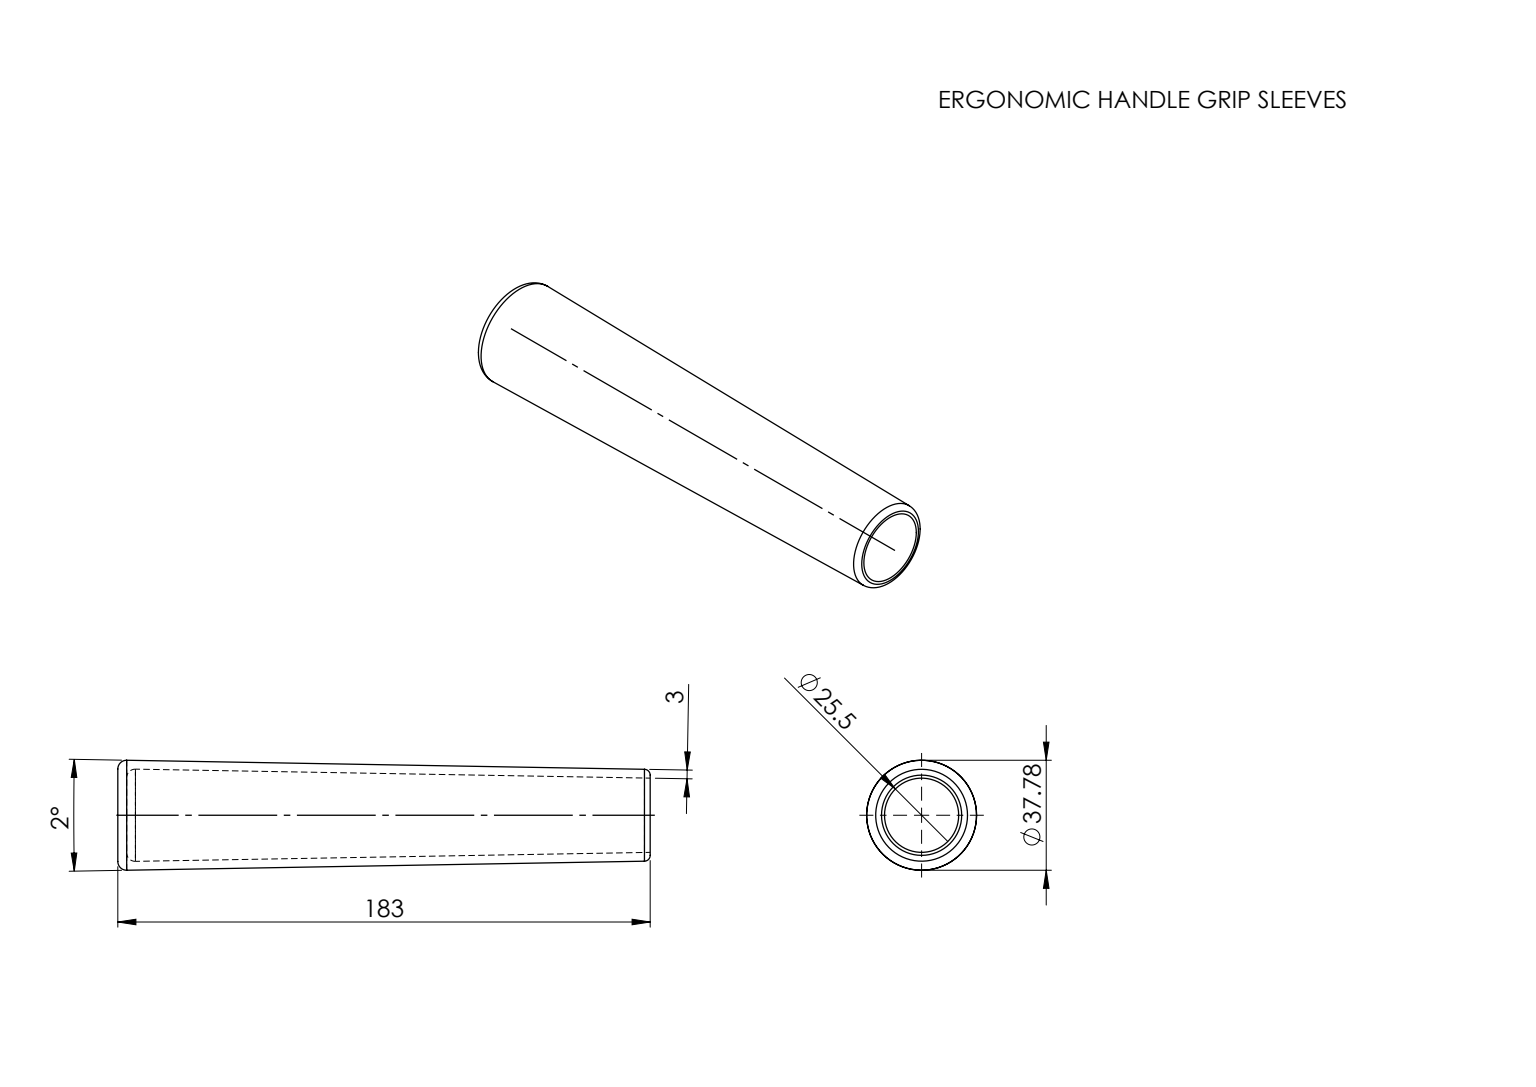
ISO-10303-21;
HEADER;
FILE_DESCRIPTION (('STEP AP214'),
    '1' );
FILE_NAME ('Ergonomic Handle Grip Sleeves.step',
    '2026-10-02T13:02:33',
    ( '' ),
    ( '' ),
    'SwSTEP 2.0',
    'SolidWorks 2026',
    '' );
FILE_SCHEMA (( 'AUTOMOTIVE_DESIGN' ));
ENDSEC;

DATA;
#12=AXIS2_PLACEMENT_3D ( 'NONE', #5144, #6683, #9508 ) ;
#70=( NAMED_UNIT ( * ) SI_UNIT ( $, .STERADIAN. ) SOLID_ANGLE_UNIT ( ) );
#80=ORIENTED_EDGE ( 'NONE', *, *, #17512, .T. ) ;
#102=ORIENTED_EDGE ( 'NONE', *, *, #16935, .T. ) ;
#181=ORIENTED_EDGE ( 'NONE', *, *, #3310, .F. ) ;
#194=( NAMED_UNIT ( * ) PLANE_ANGLE_UNIT ( ) SI_UNIT ( $, .RADIAN. ) );
#220=EDGE_CURVE ( 'NONE', #5802, #9058, #10861, .T. ) ;
#233=ORIENTED_EDGE ( 'NONE', *, *, #9764, .F. ) ;
#364=APPLICATION_CONTEXT ( 'automotive_design' ) ;
#380=CIRCLE ( 'NONE', #16419, 13.78215425775057668 ) ;
#447=DIRECTION ( 'NONE',  ( 0.000000000000000000, 0.000000000000000000, -1.000000000000000000 ) ) ;
#481=CARTESIAN_POINT ( 'NONE',  ( -131.1404785418517918, -2.850701963179328668, -13.78215425775057490 ) ) ;
#490=CIRCLE ( 'NONE', #15932, 13.78215425775057668 ) ;
#611=FACE_OUTER_BOUND ( 'NONE', #2046, .T. ) ;
#789=CARTESIAN_POINT ( 'NONE',  ( -131.1055737289773617, -2.850701963179328668, 9.951701414186818625E-16 ) ) ;
#845=ORIENTED_EDGE ( 'NONE', *, *, #9764, .T. ) ;
#922=CARTESIAN_POINT ( 'NONE',  ( -129.1404785418517918, -2.850701963179328668, 9.951701414186818625E-16 ) ) ;
#1010=ORIENTED_EDGE ( 'NONE', *, *, #8263, .T. ) ;
#1036=EDGE_LOOP ( 'NONE', ( #5576, #5988 ) ) ;
#1053=ORIENTED_EDGE ( 'NONE', *, *, #2494, .F. ) ;
#1132=VERTEX_POINT ( 'NONE', #18787 ) ;
#1237=ORIENTED_EDGE ( 'NONE', *, *, #1546, .T. ) ;
#1428=DIRECTION ( 'NONE',  ( 0.000000000000000000, 0.000000000000000000, 1.000000000000000000 ) ) ;
#1519=CARTESIAN_POINT ( 'NONE',  ( -306.0881213225399051, -2.850701963179328668, 9.951701414186818625E-16 ) ) ;
#1525=CIRCLE ( 'NONE', #11179, 18.88854657239857815 ) ;
#1546=EDGE_CURVE ( 'NONE', #6009, #3698, #17797, .T. ) ;
#1589=( NAMED_UNIT ( * ) PLANE_ANGLE_UNIT ( ) SI_UNIT ( $, .RADIAN. ) );
#1674=DIRECTION ( 'NONE',  ( -1.000000000000000000, 0.000000000000000000, 0.000000000000000000 ) ) ;
#1677=EDGE_LOOP ( 'NONE', ( #11273, #1237, #15915, #6184 ) ) ;
#1683=DIRECTION ( 'NONE',  ( 0.000000000000000000, 1.000000000000000000, -1.224646799147353207E-16 ) ) ;
#1701=ORIENTED_EDGE ( 'NONE', *, *, #4888, .T. ) ;
#1709=ORIENTED_EDGE ( 'NONE', *, *, #10798, .T. ) ;
#1812=FACE_OUTER_BOUND ( 'NONE', #16311, .T. ) ;
#1827=CIRCLE ( 'NONE', #14256, 18.88854657239857815 ) ;
#1899=UNCERTAINTY_MEASURE_WITH_UNIT (LENGTH_MEASURE( 1.000000000000000082E-05 ), #7601, 'distance_accuracy_value', 'NONE');
#1933=EDGE_CURVE ( 'NONE', #6009, #10091, #5194, .T. ) ;
#2046=EDGE_LOOP ( 'NONE', ( #7736, #9894, #11498, #9115 ) ) ;
#2058=CARTESIAN_POINT ( 'NONE',  ( -129.1404785418517918, -2.850701963179328668, 9.951701414186818625E-16 ) ) ;
#2108=CARTESIAN_POINT ( 'NONE',  ( -309.1404785418517918, -2.850701963179328668, 9.951701414186818625E-16 ) ) ;
#2162=DIRECTION ( 'NONE',  ( 0.000000000000000000, 0.000000000000000000, -1.000000000000000000 ) ) ;
#2247=DIRECTION ( 'NONE',  ( 0.000000000000000000, -1.000000000000000000, 0.000000000000000000 ) ) ;
#2480=MANIFOLD_SOLID_BREP ( 'Cavity1', #10549 ) ;
#2486=ORIENTED_EDGE ( 'NONE', *, *, #10798, .F. ) ;
#2487=ADVANCED_FACE ( 'NONE', ( #1812 ), #4558, .T. ) ;
#2489=EDGE_CURVE ( 'NONE', #6795, #5802, #5832, .T. ) ;
#2494=EDGE_CURVE ( 'NONE', #10067, #10091, #380, .T. ) ;
#2512=CARTESIAN_POINT ( 'NONE',  ( -131.1055737289773617, -2.850701963179328668, -15.78184964806336055 ) ) ;
#2533=DIRECTION ( 'NONE',  ( -1.000000000000000000, 0.000000000000000000, 0.000000000000000000 ) ) ;
#2537=VERTEX_POINT ( 'NONE', #10885 ) ;
#2720=CARTESIAN_POINT ( 'NONE',  ( -309.1404785418517918, -2.850701963179328668, 9.951701414186818625E-16 ) ) ;
#2763=VECTOR ( 'NONE', #3525, 1000.000000000000114 ) ;
#2778=CARTESIAN_POINT ( 'NONE',  ( -129.1404785418517918, -2.850701963179326892, -12.74754878398196389 ) ) ;
#2882=EDGE_CURVE ( 'NONE', #3698, #9058, #7770, .T. ) ;
#2886=( NAMED_UNIT ( * ) SI_UNIT ( $, .STERADIAN. ) SOLID_ANGLE_UNIT ( ) );
#2950=EDGE_LOOP ( 'NONE', ( #7070, #12584, #14818, #11398 ) ) ;
#2982=FACE_OUTER_BOUND ( 'NONE', #15483, .T. ) ;
#3054=CARTESIAN_POINT ( 'NONE',  ( -129.1404785418517918, -2.850701963179328668, 9.951701414186818625E-16 ) ) ;
#3061=ADVANCED_FACE ( 'NONE', ( #11418 ), #3510, .T. ) ;
#3149=ORIENTED_EDGE ( 'NONE', *, *, #17512, .F. ) ;
#3162=DIRECTION ( 'NONE',  ( -1.000000000000000000, 0.000000000000000000, 0.000000000000000000 ) ) ;
#3182=DIRECTION ( 'NONE',  ( -0.9998476951563911586, 0.000000000000000000, 0.01745240643728354635 ) ) ;
#3210=PRESENTATION_STYLE_ASSIGNMENT (( #14519 ) ) ;
#3227=VERTEX_POINT ( 'NONE', #4413 ) ;
#3262=CONICAL_SURFACE ( 'NONE', #5717, 15.74754878398195856, 0.01745329251994333364 ) ;
#3285=CARTESIAN_POINT ( 'NONE',  ( -129.1404785418517918, -2.850701963179328668, 9.951701414186818625E-16 ) ) ;
#3310=EDGE_CURVE ( 'NONE', #2537, #8740, #16558, .T. ) ;
#3339=CARTESIAN_POINT ( 'NONE',  ( -129.1404785418517918, -2.850701963179328668, 9.951701414186818625E-16 ) ) ;
#3365=AXIS2_PLACEMENT_3D ( 'NONE', #3054, #11477, #14434 ) ;
#3397=CARTESIAN_POINT ( 'NONE',  ( -129.1404785418517918, -2.850701963179328668, 9.951701414186818625E-16 ) ) ;
#3510=TOROIDAL_SURFACE ( 'NONE', #12607, 13.78215425775057668, 2.000000000000000000 ) ;
#3525=DIRECTION ( 'NONE',  ( -0.9998476951563911586, -2.137303368083795934E-18, 0.01745240643728354635 ) ) ;
#3566=ORIENTED_EDGE ( 'NONE', *, *, #18340, .F. ) ;
#3571=CARTESIAN_POINT ( 'NONE',  ( -312.1404785418517918, -2.850701963179328668, 15.88900348692940945 ) ) ;
#3616=CONICAL_SURFACE ( 'NONE', #14826, 12.74754878398196567, 0.01745329251994333364 ) ;
#3698=VERTEX_POINT ( 'NONE', #6213 ) ;
#3713=CARTESIAN_POINT ( 'NONE',  ( -309.1404785418517918, -2.850701963179328668, 9.951701414186818625E-16 ) ) ;
#3936=PRODUCT ( 'Ergonomic Handle Grip Sleeves', 'Ergonomic Handle Grip Sleeves', '', ( #17404 ) ) ;
#4038=ADVANCED_FACE ( 'NONE', ( #11937 ), #3616, .F. ) ;
#4042=EDGE_CURVE ( 'NONE', #10626, #3227, #8172, .T. ) ;
#4073=ORIENTED_EDGE ( 'NONE', *, *, #9817, .T. ) ;
#4106=DIRECTION ( 'NONE',  ( 0.000000000000000000, 0.000000000000000000, -1.000000000000000000 ) ) ;
#4113=AXIS2_PLACEMENT_3D ( 'NONE', #14799, #7611, #12017 ) ;
#4153=DIRECTION ( 'NONE',  ( -1.000000000000000000, 0.000000000000000000, 0.000000000000000000 ) ) ;
#4207=EDGE_CURVE ( 'NONE', #6795, #3698, #1827, .T. ) ;
#4223=SURFACE_STYLE_FILL_AREA ( #9827 ) ;
#4381=DIRECTION ( 'NONE',  ( 0.000000000000000000, 1.000000000000000000, 1.224646799147353207E-16 ) ) ;
#4413=CARTESIAN_POINT ( 'NONE',  ( -309.1404785418517918, -2.850701963179328668, 12.83663829214476237 ) ) ;
#4435=CARTESIAN_POINT ( 'NONE',  ( -306.0881213225399051, -2.850701963179328668, 9.951701414186818625E-16 ) ) ;
#4438=EDGE_LOOP ( 'NONE', ( #10812, #3149, #8903, #13669 ) ) ;
#4457=( NAMED_UNIT ( * ) SI_UNIT ( $, .STERADIAN. ) SOLID_ANGLE_UNIT ( ) );
#4558=PLANE ( 'NONE',  #17659 ) ;
#4619=LINE ( 'NONE', #14587, #5735 ) ;
#4743=AXIS2_PLACEMENT_3D ( 'NONE', #922, #14549, #15784 ) ;
#4759=DIRECTION ( 'NONE',  ( -1.000000000000000000, 0.000000000000000000, 0.000000000000000000 ) ) ;
#4774=CARTESIAN_POINT ( 'NONE',  ( -129.1404785418517918, -2.850701963179330445, 15.74754878398195856 ) ) ;
#4860=DIRECTION ( 'NONE',  ( 0.000000000000000000, 0.000000000000000000, -1.000000000000000000 ) ) ;
#4888=EDGE_CURVE ( 'NONE', #10626, #1132, #9354, .T. ) ;
#4891=MECHANICAL_DESIGN_GEOMETRIC_PRESENTATION_REPRESENTATION('',(#7057),#11847);
#4896=FACE_OUTER_BOUND ( 'NONE', #1036, .T. ) ;
#5144=CARTESIAN_POINT ( 'NONE',  ( -306.1404785418517918, -2.850701963179328668, 12.83663829214476237 ) ) ;
#5194=CIRCLE ( 'NONE', #16084, 1.999999999999998224 ) ;
#5392=AXIS2_PLACEMENT_3D ( 'NONE', #481, #14785, #16496 ) ;
#5484=DIRECTION ( 'NONE',  ( 1.000000000000000000, 0.000000000000000000, 0.000000000000000000 ) ) ;
#5576=ORIENTED_EDGE ( 'NONE', *, *, #2494, .T. ) ;
#5579=EDGE_LOOP ( 'NONE', ( #6921, #11878, #1053, #3566 ) ) ;
#5717=AXIS2_PLACEMENT_3D ( 'NONE', #11863, #10452, #4860 ) ;
#5735=VECTOR ( 'NONE', #3182, 1000.000000000000114 ) ;
#5768=FILL_AREA_STYLE_COLOUR ( '', #11989 ) ;
#5800=DIRECTION ( 'NONE',  ( 1.000000000000000000, -0.000000000000000000, -0.000000000000000000 ) ) ;
#5802=VERTEX_POINT ( 'NONE', #12430 ) ;
#5832=CIRCLE ( 'NONE', #16737, 2.999999999999999112 ) ;
#5853=SHAPE_REPRESENTATION_RELATIONSHIP ( 'NONE' , 'NONE' ,  #13723, #9123 ) ;
#5906=ORIENTED_EDGE ( 'NONE', *, *, #11599, .F. ) ;
#5914=DIRECTION ( 'NONE',  ( 0.000000000000000000, 0.000000000000000000, -1.000000000000000000 ) ) ;
#5950=DIRECTION ( 'NONE',  ( 0.000000000000000000, 2.168404344971010840E-16, 1.000000000000000000 ) ) ;
#5988=ORIENTED_EDGE ( 'NONE', *, *, #14498, .T. ) ;
#6009=VERTEX_POINT ( 'NONE', #9705 ) ;
#6056=CARTESIAN_POINT ( 'NONE',  ( -309.1404785418517918, -2.850701963179326892, -12.83663829214475882 ) ) ;
#6078=AXIS2_PLACEMENT_3D ( 'NONE', #6729, #1674, #13131 ) ;
#6183=DIRECTION ( 'NONE',  ( -1.000000000000000000, 0.000000000000000000, 0.000000000000000000 ) ) ;
#6184=ORIENTED_EDGE ( 'NONE', *, *, #14460, .F. ) ;
#6213=CARTESIAN_POINT ( 'NONE',  ( -309.0881213225398483, -2.850701963179330889, 18.88854657239857815 ) ) ;
#6225=ADVANCED_FACE ( 'NONE', ( #7219 ), #16851, .F. ) ;
#6309=DIRECTION ( 'NONE',  ( 0.000000000000000000, 0.000000000000000000, 1.000000000000000000 ) ) ;
#6392=CIRCLE ( 'NONE', #11777, 15.78184964806336055 ) ;
#6478=ORIENTED_EDGE ( 'NONE', *, *, #16016, .T. ) ;
#6493=ADVANCED_FACE ( 'NONE', ( #10339 ), #14711, .T. ) ;
#6580=EDGE_LOOP ( 'NONE', ( #2486, #233 ) ) ;
#6640=AXIS2_PLACEMENT_3D ( 'NONE', #4435, #5800, #15911 ) ;
#6683=DIRECTION ( 'NONE',  ( 0.000000000000000000, -1.000000000000000000, 0.000000000000000000 ) ) ;
#6689=DIRECTION ( 'NONE',  ( 0.000000000000000000, 0.000000000000000000, 1.000000000000000000 ) ) ;
#6728=CARTESIAN_POINT ( 'NONE',  ( -131.1404785418517918, -2.850701963179328668, 9.951701414186818625E-16 ) ) ;
#6729=CARTESIAN_POINT ( 'NONE',  ( -312.1404785418517918, -2.850701963179328668, 9.951701414186818625E-16 ) ) ;
#6795=VERTEX_POINT ( 'NONE', #8722 ) ;
#6814=CARTESIAN_POINT ( 'NONE',  ( -129.1404785418517918, -2.850701963179328668, 9.951701414186818625E-16 ) ) ;
#6921=ORIENTED_EDGE ( 'NONE', *, *, #8263, .F. ) ;
#7057=STYLED_ITEM ( 'NONE', ( #3210 ), #2480 ) ;
#7070=ORIENTED_EDGE ( 'NONE', *, *, #1933, .F. ) ;
#7106=DIRECTION ( 'NONE',  ( 0.000000000000000000, 0.000000000000000000, 1.000000000000000000 ) ) ;
#7219=FACE_OUTER_BOUND ( 'NONE', #8816, .T. ) ;
#7268=AXIS2_PLACEMENT_3D ( 'NONE', #3285, #14772, #11628 ) ;
#7473=DIRECTION ( 'NONE',  ( 0.000000000000000000, 0.000000000000000000, 1.000000000000000000 ) ) ;
#7523=DIRECTION ( 'NONE',  ( 1.000000000000000000, -0.000000000000000000, -0.000000000000000000 ) ) ;
#7543=ADVANCED_FACE ( 'NONE', ( #10153 ), #16110, .T. ) ;
#7550=CONICAL_SURFACE ( 'NONE', #9055, 12.74754878398196567, 0.01745329251994333364 ) ;
#7601=( LENGTH_UNIT ( ) NAMED_UNIT ( * ) SI_UNIT ( .MILLI., .METRE. ) );
#7611=DIRECTION ( 'NONE',  ( 1.000000000000000000, 0.000000000000000000, 0.000000000000000000 ) ) ;
#7727=DIRECTION ( 'NONE',  ( 0.000000000000000000, 0.000000000000000000, 1.000000000000000000 ) ) ;
#7736=ORIENTED_EDGE ( 'NONE', *, *, #4207, .F. ) ;
#7749=DIRECTION ( 'NONE',  ( 1.000000000000000000, 0.000000000000000000, 0.000000000000000000 ) ) ;
#7770=CIRCLE ( 'NONE', #11721, 2.999999999999999112 ) ;
#7979=ORIENTED_EDGE ( 'NONE', *, *, #220, .T. ) ;
#8050=DIRECTION ( 'NONE',  ( 0.000000000000000000, -1.445602896647339656E-16, 1.000000000000000000 ) ) ;
#8115=CIRCLE ( 'NONE', #17563, 12.83663829214476060 ) ;
#8172=CIRCLE ( 'NONE', #12, 3.000000000000000888 ) ;
#8203=ORIENTED_EDGE ( 'NONE', *, *, #15252, .F. ) ;
#8263=EDGE_CURVE ( 'NONE', #6009, #14985, #9591, .T. ) ;
#8323=DIRECTION ( 'NONE',  ( 0.000000000000000000, 0.000000000000000000, -1.000000000000000000 ) ) ;
#8404=SURFACE_STYLE_USAGE ( .BOTH. , #15883 ) ;
#8524=CIRCLE ( 'NONE', #17934, 12.83663829214476060 ) ;
#8594=CARTESIAN_POINT ( 'NONE',  ( -309.1404785418517918, -2.850701963179328668, 9.951701414186818625E-16 ) ) ;
#8664=CARTESIAN_POINT ( 'NONE',  ( -306.1404785418517918, -2.850701963179328668, 9.951701414186818625E-16 ) ) ;
#8670=EDGE_LOOP ( 'NONE', ( #17913, #17680, #18762, #1709 ) ) ;
#8722=CARTESIAN_POINT ( 'NONE',  ( -309.0881213225398483, -2.850701963179328668, -18.88854657239857815 ) ) ;
#8740=VERTEX_POINT ( 'NONE', #15263 ) ;
#8775=AXIS2_PLACEMENT_3D ( 'NONE', #2108, #4759, #16151 ) ;
#8816=EDGE_LOOP ( 'NONE', ( #1701, #4073, #845, #11378 ) ) ;
#8903=ORIENTED_EDGE ( 'NONE', *, *, #11599, .T. ) ;
#8944=FACE_OUTER_BOUND ( 'NONE', #17638, .T. ) ;
#8996=FACE_OUTER_BOUND ( 'NONE', #8670, .T. ) ;
#8999=PRODUCT_DEFINITION_FORMATION_WITH_SPECIFIED_SOURCE ( 'ANY', '', #3936, .NOT_KNOWN. ) ;
#9003=CARTESIAN_POINT ( 'NONE',  ( -312.1404785418517918, -2.850701963179328668, 9.951701414186818625E-16 ) ) ;
#9055=AXIS2_PLACEMENT_3D ( 'NONE', #10183, #3162, #11413 ) ;
#9058=VERTEX_POINT ( 'NONE', #3571 ) ;
#9070=DIRECTION ( 'NONE',  ( -1.000000000000000000, -0.000000000000000000, -0.000000000000000000 ) ) ;
#9115=ORIENTED_EDGE ( 'NONE', *, *, #2882, .F. ) ;
#9123=ADVANCED_BREP_SHAPE_REPRESENTATION ( '', ( #2480, #18772 ), #9301 ) ;
#9170=CARTESIAN_POINT ( 'NONE',  ( -131.1055737289773617, -2.850701963179328668, 9.951701414186818625E-16 ) ) ;
#9204=DIRECTION ( 'NONE',  ( 0.000000000000000000, 1.000000000000000000, 1.224646799147353207E-16 ) ) ;
#9259=CARTESIAN_POINT ( 'NONE',  ( -129.1404785418517918, -2.850701963179328668, -15.74754878398195856 ) ) ;
#9301=( GEOMETRIC_REPRESENTATION_CONTEXT ( 3 ) GLOBAL_UNCERTAINTY_ASSIGNED_CONTEXT ( ( #11907 ) ) GLOBAL_UNIT_ASSIGNED_CONTEXT ( ( #13122, #12930, #2886 ) ) REPRESENTATION_CONTEXT ( 'NONE', 'WORKASPACE' ) );
#9354=CIRCLE ( 'NONE', #6640, 15.83618137761393463 ) ;
#9508=DIRECTION ( 'NONE',  ( 0.000000000000000000, 0.000000000000000000, -1.000000000000000000 ) ) ;
#9591=CIRCLE ( 'NONE', #17184, 15.78184964806336055 ) ;
#9659=FACE_OUTER_BOUND ( 'NONE', #9756, .T. ) ;
#9705=CARTESIAN_POINT ( 'NONE',  ( -131.1055737289773617, -2.850701963179330445, 15.78184964806336055 ) ) ;
#9756=EDGE_LOOP ( 'NONE', ( #18372, #8203, #16661, #17766 ) ) ;
#9764=EDGE_CURVE ( 'NONE', #10224, #3227, #8524, .T. ) ;
#9817=EDGE_CURVE ( 'NONE', #1132, #10224, #16435, .T. ) ;
#9827=FILL_AREA_STYLE ('',( #5768 ) ) ;
#9878=CARTESIAN_POINT ( 'NONE',  ( -306.1404785418517918, -2.850701963179326892, -12.83663829214475882 ) ) ;
#9894=ORIENTED_EDGE ( 'NONE', *, *, #2489, .T. ) ;
#9940=DIRECTION ( 'NONE',  ( 0.000000000000000000, 0.000000000000000000, 1.000000000000000000 ) ) ;
#10067=VERTEX_POINT ( 'NONE', #16588 ) ;
#10091=VERTEX_POINT ( 'NONE', #15059 ) ;
#10153=FACE_OUTER_BOUND ( 'NONE', #1677, .T. ) ;
#10183=CARTESIAN_POINT ( 'NONE',  ( -129.1404785418517918, -2.850701963179328668, 9.951701414186818625E-16 ) ) ;
#10198=STYLED_ITEM ( 'NONE', ( #12753 ), #9123 ) ;
#10224=VERTEX_POINT ( 'NONE', #6056 ) ;
#10232=UNCERTAINTY_MEASURE_WITH_UNIT (LENGTH_MEASURE( 1.000000000000000082E-05 ), #18607, 'distance_accuracy_value', 'NONE');
#10339=FACE_OUTER_BOUND ( 'NONE', #2950, .T. ) ;
#10345=DIRECTION ( 'NONE',  ( -1.000000000000000000, 0.000000000000000000, 0.000000000000000000 ) ) ;
#10413=PRODUCT_DEFINITION_CONTEXT ( 'detailed design', #11355, 'design' ) ;
#10452=DIRECTION ( 'NONE',  ( -1.000000000000000000, -0.000000000000000000, -0.000000000000000000 ) ) ;
#10484=DIRECTION ( 'NONE',  ( 0.000000000000000000, 0.000000000000000000, -1.000000000000000000 ) ) ;
#10549=CLOSED_SHELL ( 'NONE', ( #6225, #12001, #3061, #12616, #7543, #11856, #2487, #16720, #17958, #6493, #4038, #11913, #11206 ) ) ;
#10590=LINE ( 'NONE', #9259, #17764 ) ;
#10626=VERTEX_POINT ( 'NONE', #14083 ) ;
#10798=EDGE_CURVE ( 'NONE', #3227, #10224, #8115, .T. ) ;
#10812=ORIENTED_EDGE ( 'NONE', *, *, #16935, .F. ) ;
#10861=CIRCLE ( 'NONE', #12675, 15.88900348692940945 ) ;
#10885=CARTESIAN_POINT ( 'NONE',  ( -129.1404785418517918, -2.850701963179326892, -12.74754878398196389 ) ) ;
#11154=VECTOR ( 'NONE', #15936, 1000.000000000000114 ) ;
#11179=AXIS2_PLACEMENT_3D ( 'NONE', #14906, #7523, #5914 ) ;
#11187=DIRECTION ( 'NONE',  ( 0.000000000000000000, 0.000000000000000000, -1.000000000000000000 ) ) ;
#11205=PRODUCT_DEFINITION_SHAPE ( 'NONE', 'NONE',  #12169 ) ;
#11206=ADVANCED_FACE ( 'NONE', ( #8996 ), #15371, .F. ) ;
#11273=ORIENTED_EDGE ( 'NONE', *, *, #12839, .T. ) ;
#11355=APPLICATION_CONTEXT ( 'automotive_design' ) ;
#11378=ORIENTED_EDGE ( 'NONE', *, *, #4042, .F. ) ;
#11398=ORIENTED_EDGE ( 'NONE', *, *, #14498, .F. ) ;
#11402=MECHANICAL_DESIGN_GEOMETRIC_PRESENTATION_REPRESENTATION('',(#10198),#16579);
#11413=DIRECTION ( 'NONE',  ( 0.000000000000000000, 0.000000000000000000, 1.000000000000000000 ) ) ;
#11418=FACE_OUTER_BOUND ( 'NONE', #5579, .T. ) ;
#11450=CIRCLE ( 'NONE', #15403, 15.83618137761393463 ) ;
#11458=CIRCLE ( 'NONE', #7268, 12.74754878398196567 ) ;
#11477=DIRECTION ( 'NONE',  ( -1.000000000000000000, -0.000000000000000000, -0.000000000000000000 ) ) ;
#11498=ORIENTED_EDGE ( 'NONE', *, *, #16016, .F. ) ;
#11599=EDGE_CURVE ( 'NONE', #8740, #10626, #4619, .T. ) ;
#11628=DIRECTION ( 'NONE',  ( 0.000000000000000000, 0.000000000000000000, -1.000000000000000000 ) ) ;
#11636=EDGE_CURVE ( 'NONE', #1132, #10626, #11450, .T. ) ;
#11638=FILL_AREA_STYLE ('',( #14787 ) ) ;
#11721=AXIS2_PLACEMENT_3D ( 'NONE', #16679, #2247, #2162 ) ;
#11777=AXIS2_PLACEMENT_3D ( 'NONE', #789, #13945, #11187 ) ;
#11784=ORIENTED_EDGE ( 'NONE', *, *, #4207, .T. ) ;
#11847=( GEOMETRIC_REPRESENTATION_CONTEXT ( 3 ) GLOBAL_UNCERTAINTY_ASSIGNED_CONTEXT ( ( #1899 ) ) GLOBAL_UNIT_ASSIGNED_CONTEXT ( ( #7601, #194, #4457 ) ) REPRESENTATION_CONTEXT ( 'NONE', 'WORKASPACE' ) );
#11856=ADVANCED_FACE ( 'NONE', ( #4896, #12182 ), #16780, .T. ) ;
#11863=CARTESIAN_POINT ( 'NONE',  ( -129.1404785418517918, -2.850701963179328668, 9.951701414186818625E-16 ) ) ;
#11878=ORIENTED_EDGE ( 'NONE', *, *, #1933, .T. ) ;
#11907=UNCERTAINTY_MEASURE_WITH_UNIT (LENGTH_MEASURE( 1.000000000000000082E-05 ), #13122, 'distance_accuracy_value', 'NONE');
#11913=ADVANCED_FACE ( 'NONE', ( #14087 ), #15693, .F. ) ;
#11914=DIRECTION ( 'NONE',  ( 0.000000000000000000, 0.000000000000000000, 1.000000000000000000 ) ) ;
#11937=FACE_OUTER_BOUND ( 'NONE', #4438, .T. ) ;
#11989=COLOUR_RGB ( '', 0.66274510, 0.83137255, 0.94901961) ;
#12001=ADVANCED_FACE ( 'NONE', ( #2982 ), #7550, .F. ) ;
#12017=DIRECTION ( 'NONE',  ( 0.000000000000000000, 0.000000000000000000, -1.000000000000000000 ) ) ;
#12018=AXIS2_PLACEMENT_3D ( 'NONE', #8664, #14265, #12826 ) ;
#12047=AXIS2_PLACEMENT_3D ( 'NONE', #6814, #12757, #17144 ) ;
#12146=COLOUR_RGB ( '', 0.66274510, 0.83137255, 0.94901961) ;
#12169=PRODUCT_DEFINITION ( 'UNKNOWN', '', #8999, #10413 ) ;
#12182=FACE_BOUND ( 'NONE', #16140, .T. ) ;
#12406=DIRECTION ( 'NONE',  ( 1.000000000000000000, 0.000000000000000000, 0.000000000000000000 ) ) ;
#12430=CARTESIAN_POINT ( 'NONE',  ( -312.1404785418517918, -2.850701963179326892, -15.88900348692940945 ) ) ;
#12482=AXIS2_PLACEMENT_3D ( 'NONE', #9878, #4381, #18570 ) ;
#12584=ORIENTED_EDGE ( 'NONE', *, *, #12839, .F. ) ;
#12607=AXIS2_PLACEMENT_3D ( 'NONE', #6728, #5484, #8323 ) ;
#12616=ADVANCED_FACE ( 'NONE', ( #611 ), #14834, .T. ) ;
#12675=AXIS2_PLACEMENT_3D ( 'NONE', #17587, #10345, #16047 ) ;
#12753=PRESENTATION_STYLE_ASSIGNMENT (( #8404 ) ) ;
#12757=DIRECTION ( 'NONE',  ( 1.000000000000000000, 0.000000000000000000, 0.000000000000000000 ) ) ;
#12826=DIRECTION ( 'NONE',  ( 0.000000000000000000, 0.000000000000000000, 1.000000000000000000 ) ) ;
#12839=EDGE_CURVE ( 'NONE', #14985, #6009, #6392, .T. ) ;
#12930=( NAMED_UNIT ( * ) PLANE_ANGLE_UNIT ( ) SI_UNIT ( $, .RADIAN. ) );
#13122=( LENGTH_UNIT ( ) NAMED_UNIT ( * ) SI_UNIT ( .MILLI., .METRE. ) );
#13131=DIRECTION ( 'NONE',  ( 0.000000000000000000, 0.000000000000000000, 1.000000000000000000 ) ) ;
#13309=DIRECTION ( 'NONE',  ( -1.000000000000000000, 0.000000000000000000, 0.000000000000000000 ) ) ;
#13365=SURFACE_SIDE_STYLE ('',( #14613 ) ) ;
#13492=ORIENTED_EDGE ( 'NONE', *, *, #4888, .F. ) ;
#13611=CARTESIAN_POINT ( 'NONE',  ( 0.000000000000000000, 0.000000000000000000, 0.000000000000000000 ) ) ;
#13669=ORIENTED_EDGE ( 'NONE', *, *, #11636, .F. ) ;
#13723=SHAPE_REPRESENTATION ( 'Ergonomic Handle Grip Sleeves', ( #18772 ), #9301 ) ;
#13945=DIRECTION ( 'NONE',  ( -1.000000000000000000, -0.000000000000000000, -0.000000000000000000 ) ) ;
#14083=CARTESIAN_POINT ( 'NONE',  ( -306.0881213225399051, -2.850701963179328668, 15.83618137761393463 ) ) ;
#14087=FACE_OUTER_BOUND ( 'NONE', #6580, .T. ) ;
#14256=AXIS2_PLACEMENT_3D ( 'NONE', #18495, #17047, #4106 ) ;
#14265=DIRECTION ( 'NONE',  ( -1.000000000000000000, 0.000000000000000000, 0.000000000000000000 ) ) ;
#14402=DIRECTION ( 'NONE',  ( 1.000000000000000000, -0.000000000000000000, -0.000000000000000000 ) ) ;
#14434=DIRECTION ( 'NONE',  ( 0.000000000000000000, 0.000000000000000000, -1.000000000000000000 ) ) ;
#14460=EDGE_CURVE ( 'NONE', #14985, #6795, #10590, .T. ) ;
#14498=EDGE_CURVE ( 'NONE', #10091, #10067, #490, .T. ) ;
#14519=SURFACE_STYLE_USAGE ( .BOTH. , #13365 ) ;
#14549=DIRECTION ( 'NONE',  ( -1.000000000000000000, -0.000000000000000000, -0.000000000000000000 ) ) ;
#14579=CARTESIAN_POINT ( 'NONE',  ( -131.1404785418517918, -2.850701963179326892, 13.78215425775057845 ) ) ;
#14587=CARTESIAN_POINT ( 'NONE',  ( -129.1404785418517918, -2.850701963179328668, 12.74754878398196745 ) ) ;
#14613=SURFACE_STYLE_FILL_AREA ( #11638 ) ;
#14711=TOROIDAL_SURFACE ( 'NONE', #4113, 13.78215425775057668, 2.000000000000000000 ) ;
#14759=DIRECTION ( 'NONE',  ( 1.000000000000000000, 0.000000000000000000, 0.000000000000000000 ) ) ;
#14772=DIRECTION ( 'NONE',  ( -1.000000000000000000, -0.000000000000000000, -0.000000000000000000 ) ) ;
#14785=DIRECTION ( 'NONE',  ( 0.000000000000000000, -1.000000000000000000, 0.000000000000000000 ) ) ;
#14787=FILL_AREA_STYLE_COLOUR ( '', #12146 ) ;
#14799=CARTESIAN_POINT ( 'NONE',  ( -131.1404785418517918, -2.850701963179328668, 9.951701414186818625E-16 ) ) ;
#14818=ORIENTED_EDGE ( 'NONE', *, *, #18340, .T. ) ;
#14826=AXIS2_PLACEMENT_3D ( 'NONE', #3339, #17890, #6309 ) ;
#14834=TOROIDAL_SURFACE ( 'NONE', #8775, 15.88900348692940945, 3.000000000000000000 ) ;
#14845=CIRCLE ( 'NONE', #6078, 15.88900348692940945 ) ;
#14906=CARTESIAN_POINT ( 'NONE',  ( -309.0881213225398483, -2.850701963179328668, 9.951701414186818625E-16 ) ) ;
#14985=VERTEX_POINT ( 'NONE', #2512 ) ;
#14991=ORIENTED_EDGE ( 'NONE', *, *, #14460, .T. ) ;
#15051=AXIS2_PLACEMENT_3D ( 'NONE', #8594, #15790, #18765 ) ;
#15059=CARTESIAN_POINT ( 'NONE',  ( -129.1404785418517918, -2.850701963179326892, 13.78215425775057845 ) ) ;
#15140=DIRECTION ( 'NONE',  ( -0.9998476951563911586, 0.000000000000000000, -0.01745240643728354635 ) ) ;
#15252=EDGE_CURVE ( 'NONE', #3698, #6795, #1525, .T. ) ;
#15263=CARTESIAN_POINT ( 'NONE',  ( -129.1404785418517918, -2.850701963179328668, 12.74754878398196745 ) ) ;
#15350=DIRECTION ( 'NONE',  ( 0.000000000000000000, 0.000000000000000000, -1.000000000000000000 ) ) ;
#15371=TOROIDAL_SURFACE ( 'NONE', #12018, 12.83663829214476060, 3.000000000000000000 ) ;
#15403=AXIS2_PLACEMENT_3D ( 'NONE', #1519, #14402, #1428 ) ;
#15483=EDGE_LOOP ( 'NONE', ( #181, #102, #13492, #5906 ) ) ;
#15681=ORIENTED_EDGE ( 'NONE', *, *, #1546, .F. ) ;
#15693=PLANE ( 'NONE',  #18453 ) ;
#15784=DIRECTION ( 'NONE',  ( 0.000000000000000000, 0.000000000000000000, -1.000000000000000000 ) ) ;
#15790=DIRECTION ( 'NONE',  ( -1.000000000000000000, 0.000000000000000000, 0.000000000000000000 ) ) ;
#15883=SURFACE_SIDE_STYLE ('',( #4223 ) ) ;
#15911=DIRECTION ( 'NONE',  ( 0.000000000000000000, 0.000000000000000000, 1.000000000000000000 ) ) ;
#15915=ORIENTED_EDGE ( 'NONE', *, *, #15252, .T. ) ;
#15932=AXIS2_PLACEMENT_3D ( 'NONE', #2058, #7749, #10484 ) ;
#15936=DIRECTION ( 'NONE',  ( -0.9998476951563911586, 2.137303368083795934E-18, -0.01745240643728354635 ) ) ;
#16016=EDGE_CURVE ( 'NONE', #9058, #5802, #14845, .T. ) ;
#16047=DIRECTION ( 'NONE',  ( 0.000000000000000000, 0.000000000000000000, 1.000000000000000000 ) ) ;
#16084=AXIS2_PLACEMENT_3D ( 'NONE', #14579, #1683, #5950 ) ;
#16110=CONICAL_SURFACE ( 'NONE', #3365, 15.74754878398195856, 0.01745329251994333364 ) ;
#16140=EDGE_LOOP ( 'NONE', ( #80, #17529 ) ) ;
#16151=DIRECTION ( 'NONE',  ( 0.000000000000000000, 0.000000000000000000, 1.000000000000000000 ) ) ;
#16311=EDGE_LOOP ( 'NONE', ( #6478, #7979 ) ) ;
#16419=AXIS2_PLACEMENT_3D ( 'NONE', #3397, #12406, #15350 ) ;
#16435=CIRCLE ( 'NONE', #12482, 3.000000000000000888 ) ;
#16455=CARTESIAN_POINT ( 'NONE',  ( -309.1404785418517918, -2.850701963179328668, 9.951701414186818625E-16 ) ) ;
#16496=DIRECTION ( 'NONE',  ( 0.000000000000000000, 0.000000000000000000, -1.000000000000000000 ) ) ;
#16558=CIRCLE ( 'NONE', #4743, 12.74754878398196567 ) ;
#16579=( GEOMETRIC_REPRESENTATION_CONTEXT ( 3 ) GLOBAL_UNCERTAINTY_ASSIGNED_CONTEXT ( ( #10232 ) ) GLOBAL_UNIT_ASSIGNED_CONTEXT ( ( #18607, #1589, #70 ) ) REPRESENTATION_CONTEXT ( 'NONE', 'WORKASPACE' ) );
#16588=CARTESIAN_POINT ( 'NONE',  ( -129.1404785418517918, -2.850701963179328668, -13.78215425775057490 ) ) ;
#16661=ORIENTED_EDGE ( 'NONE', *, *, #2882, .T. ) ;
#16679=CARTESIAN_POINT ( 'NONE',  ( -309.1404785418517918, -2.850701963179328668, 15.88900348692940945 ) ) ;
#16720=ADVANCED_FACE ( 'NONE', ( #8944 ), #3262, .T. ) ;
#16737=AXIS2_PLACEMENT_3D ( 'NONE', #17760, #9204, #8050 ) ;
#16780=PLANE ( 'NONE',  #12047 ) ;
#16851=TOROIDAL_SURFACE ( 'NONE', #17454, 12.83663829214476060, 3.000000000000000000 ) ;
#16926=DIRECTION ( 'NONE',  ( -1.000000000000000000, 0.000000000000000000, 0.000000000000000000 ) ) ;
#16935=EDGE_CURVE ( 'NONE', #2537, #1132, #17391, .T. ) ;
#17035=SHAPE_DEFINITION_REPRESENTATION ( #11205, #13723 ) ;
#17047=DIRECTION ( 'NONE',  ( 1.000000000000000000, -0.000000000000000000, -0.000000000000000000 ) ) ;
#17144=DIRECTION ( 'NONE',  ( 0.000000000000000000, 0.000000000000000000, -1.000000000000000000 ) ) ;
#17172=CARTESIAN_POINT ( 'NONE',  ( -306.1404785418517918, -2.850701963179328668, 9.951701414186818625E-16 ) ) ;
#17184=AXIS2_PLACEMENT_3D ( 'NONE', #9170, #9070, #447 ) ;
#17221=CIRCLE ( 'NONE', #5392, 2.000000000000001776 ) ;
#17391=LINE ( 'NONE', #2778, #11154 ) ;
#17404=PRODUCT_CONTEXT ( 'NONE', #364, 'mechanical' ) ;
#17454=AXIS2_PLACEMENT_3D ( 'NONE', #17172, #4153, #9940 ) ;
#17502=TOROIDAL_SURFACE ( 'NONE', #15051, 15.88900348692940945, 3.000000000000000000 ) ;
#17512=EDGE_CURVE ( 'NONE', #8740, #2537, #11458, .T. ) ;
#17529=ORIENTED_EDGE ( 'NONE', *, *, #3310, .T. ) ;
#17563=AXIS2_PLACEMENT_3D ( 'NONE', #16455, #13309, #7727 ) ;
#17587=CARTESIAN_POINT ( 'NONE',  ( -312.1404785418517918, -2.850701963179328668, 9.951701414186818625E-16 ) ) ;
#17638=EDGE_LOOP ( 'NONE', ( #15681, #1010, #14991, #11784 ) ) ;
#17659=AXIS2_PLACEMENT_3D ( 'NONE', #9003, #6183, #11914 ) ;
#17680=ORIENTED_EDGE ( 'NONE', *, *, #11636, .T. ) ;
#17760=CARTESIAN_POINT ( 'NONE',  ( -309.1404785418517918, -2.850701963179326892, -15.88900348692940945 ) ) ;
#17764=VECTOR ( 'NONE', #15140, 1000.000000000000114 ) ;
#17766=ORIENTED_EDGE ( 'NONE', *, *, #220, .F. ) ;
#17797=LINE ( 'NONE', #4774, #2763 ) ;
#17890=DIRECTION ( 'NONE',  ( -1.000000000000000000, 0.000000000000000000, 0.000000000000000000 ) ) ;
#17913=ORIENTED_EDGE ( 'NONE', *, *, #9817, .F. ) ;
#17934=AXIS2_PLACEMENT_3D ( 'NONE', #3713, #16926, #6689 ) ;
#17958=ADVANCED_FACE ( 'NONE', ( #9659 ), #17502, .T. ) ;
#18340=EDGE_CURVE ( 'NONE', #14985, #10067, #17221, .T. ) ;
#18372=ORIENTED_EDGE ( 'NONE', *, *, #2489, .F. ) ;
#18453=AXIS2_PLACEMENT_3D ( 'NONE', #2720, #2533, #7106 ) ;
#18495=CARTESIAN_POINT ( 'NONE',  ( -309.0881213225398483, -2.850701963179328668, 9.951701414186818625E-16 ) ) ;
#18570=DIRECTION ( 'NONE',  ( 0.000000000000000000, -1.445602896647338917E-16, 1.000000000000000000 ) ) ;
#18607=( LENGTH_UNIT ( ) NAMED_UNIT ( * ) SI_UNIT ( .MILLI., .METRE. ) );
#18762=ORIENTED_EDGE ( 'NONE', *, *, #4042, .T. ) ;
#18765=DIRECTION ( 'NONE',  ( 0.000000000000000000, 0.000000000000000000, 1.000000000000000000 ) ) ;
#18772=AXIS2_PLACEMENT_3D ( 'NONE', #13611, #7473, #14759 ) ;
#18787=CARTESIAN_POINT ( 'NONE',  ( -306.0881213225399051, -2.850701963179326448, -15.83618137761393463 ) ) ;
ENDSEC;
END-ISO-10303-21;
